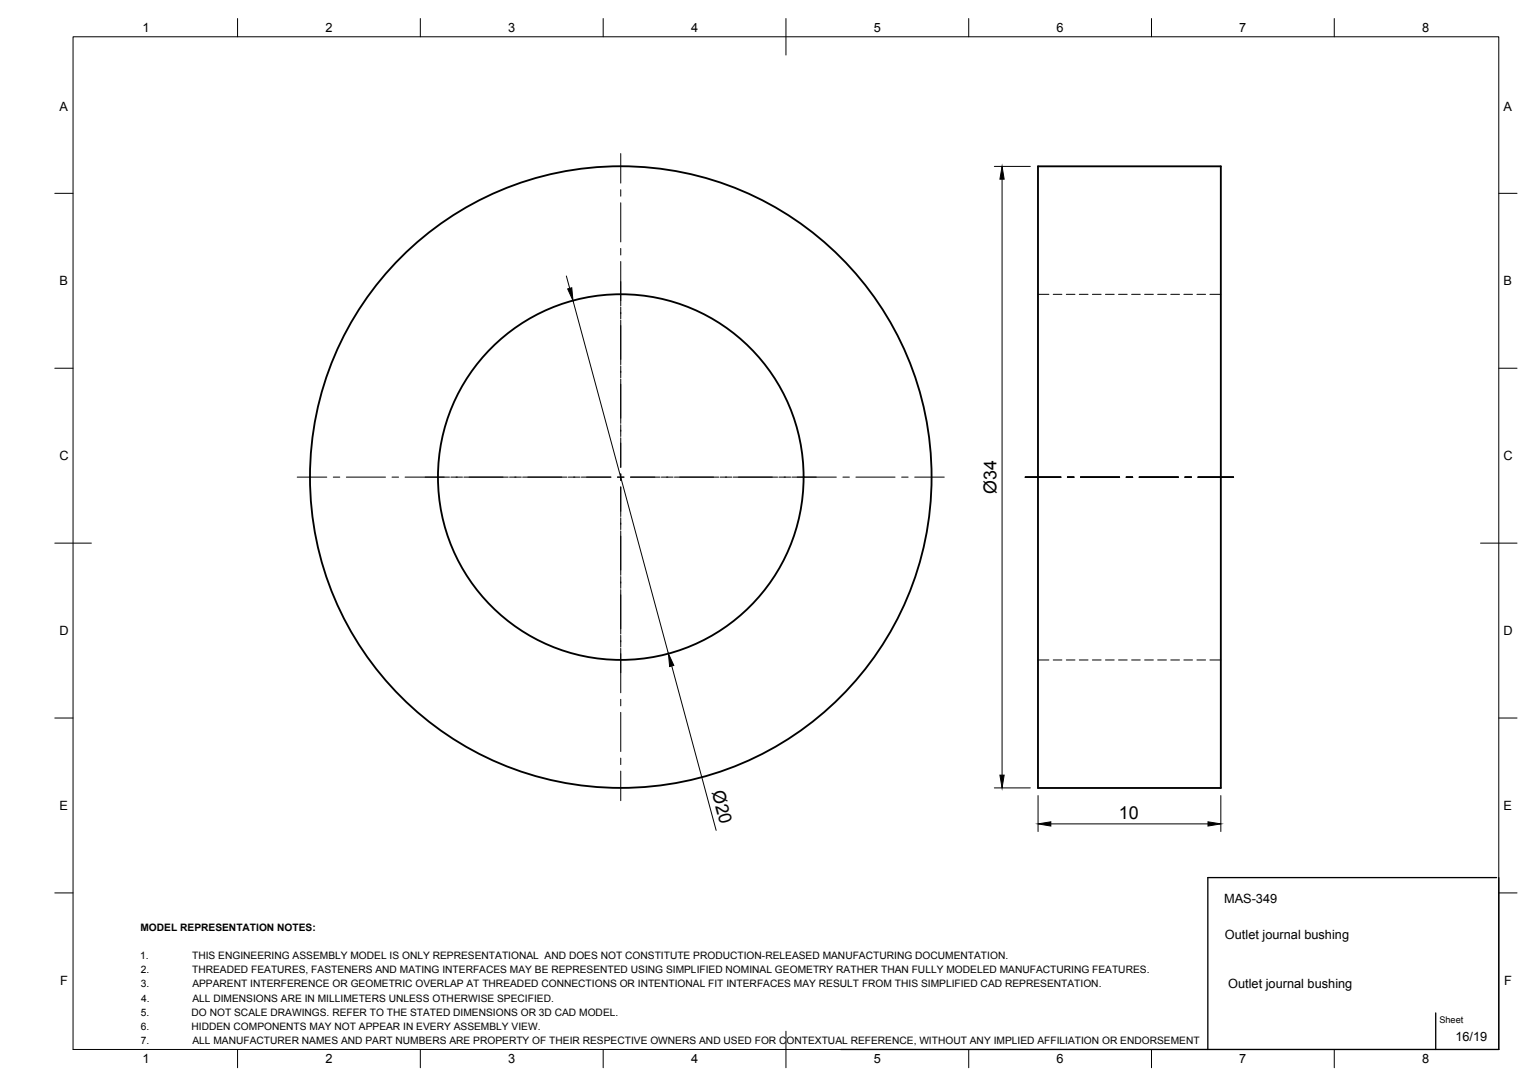
ISO-10303-21;
HEADER;
/* Generated by software containing ST-Developer
 * from STEP Tools, Inc. (www.steptools.com) 
 */

FILE_DESCRIPTION(
/* description */ ('Independent two-stage semi-open centrifugal-pump CAD. Shared impeller
s, open-machinable return casings, removable diaphragms, bronze wear/j
ournal rings, volume-preserving seal instances, retained keyed shaft, 
opposed mechanical face rings and partly threaded tie hardware. Native
 shaft rotation. Geometric topology/clearance only; flow/head/efficien
cy, pressure, cavitation, balance, preload, face loading and secondary
 seal fits/bonds, material/thermal/tolerance selection and life unassi
gned. External drive, coupling, anchors and piping bolts omitted.'),
/* implementation_level */ '2;1');

FILE_NAME(
/* name */ 'Outlet journal bushing.step',
/* time_stamp */ '2026-11-08T18:06:32-08:00',
/* author */ (''),
/* organization */ (''),
/* preprocessor_version */ 'ST-DEVELOPER v20.2',
/* originating_system */ 'Autodesk Translation Framework v15.17.0.0',
/* authorisation */ '');

FILE_SCHEMA (('AUTOMOTIVE_DESIGN { 1 0 10303 214 3 1 1 }'));
ENDSEC;

DATA;
#10=MECHANICAL_DESIGN_GEOMETRIC_PRESENTATION_REPRESENTATION('',(#406),#16687);
#368=SHAPE_REPRESENTATION_RELATIONSHIP('SRR','None',#16777,#387);
#387=ADVANCED_BREP_SHAPE_REPRESENTATION('',(#425),#16681);
#406=STYLED_ITEM('',(#16875),#425);
#425=MANIFOLD_SOLID_BREP('Body1',#6125);
#543=FACE_BOUND('',#1442,.T.);
#544=FACE_BOUND('',#1444,.T.);
#663=PLANE('',#6878);
#664=PLANE('',#6879);
#980=FACE_OUTER_BOUND('',#1439,.T.);
#981=FACE_OUTER_BOUND('',#1440,.T.);
#982=FACE_OUTER_BOUND('',#1441,.T.);
#983=FACE_OUTER_BOUND('',#1443,.T.);
#1439=EDGE_LOOP('',(#5329,#5330,#5331,#5332));
#1440=EDGE_LOOP('',(#5333,#5334,#5335,#5336));
#1441=EDGE_LOOP('',(#5337));
#1442=EDGE_LOOP('',(#5338));
#1443=EDGE_LOOP('',(#5339));
#1444=EDGE_LOOP('',(#5340));
#1820=LINE('',#15192,#2189);
#1821=LINE('',#15198,#2190);
#2189=VECTOR('',#8372,1.);
#2190=VECTOR('',#8379,1.7);
#2470=CIRCLE('',#6873,1.);
#2471=CIRCLE('',#6874,1.);
#2472=CIRCLE('',#6876,1.7);
#2473=CIRCLE('',#6877,1.7);
#2977=VERTEX_POINT('',#15189);
#2978=VERTEX_POINT('',#15191);
#2979=VERTEX_POINT('',#15195);
#2980=VERTEX_POINT('',#15197);
#3774=EDGE_CURVE('',#2977,#2977,#2470,.T.);
#3775=EDGE_CURVE('',#2977,#2978,#1820,.T.);
#3776=EDGE_CURVE('',#2978,#2978,#2471,.T.);
#3777=EDGE_CURVE('',#2979,#2979,#2472,.T.);
#3778=EDGE_CURVE('',#2979,#2980,#1821,.T.);
#3779=EDGE_CURVE('',#2980,#2980,#2473,.T.);
#5329=ORIENTED_EDGE('',*,*,#3774,.F.);
#5330=ORIENTED_EDGE('',*,*,#3775,.T.);
#5331=ORIENTED_EDGE('',*,*,#3776,.T.);
#5332=ORIENTED_EDGE('',*,*,#3775,.F.);
#5333=ORIENTED_EDGE('',*,*,#3777,.F.);
#5334=ORIENTED_EDGE('',*,*,#3778,.T.);
#5335=ORIENTED_EDGE('',*,*,#3779,.T.);
#5336=ORIENTED_EDGE('',*,*,#3778,.F.);
#5337=ORIENTED_EDGE('',*,*,#3777,.T.);
#5338=ORIENTED_EDGE('',*,*,#3774,.T.);
#5339=ORIENTED_EDGE('',*,*,#3779,.F.);
#5340=ORIENTED_EDGE('',*,*,#3776,.F.);
#5738=CYLINDRICAL_SURFACE('',#6872,1.);
#5739=CYLINDRICAL_SURFACE('',#6875,1.7);
#6059=ADVANCED_FACE('',(#980),#5738,.F.);
#6060=ADVANCED_FACE('',(#981),#5739,.T.);
#6061=ADVANCED_FACE('',(#982,#543),#663,.T.);
#6062=ADVANCED_FACE('',(#983,#544),#664,.F.);
#6125=CLOSED_SHELL('',(#6059,#6060,#6061,#6062));
#6871=AXIS2_PLACEMENT_3D('',#15187,#8366,#8367);
#6872=AXIS2_PLACEMENT_3D('',#15188,#8368,#8369);
#6873=AXIS2_PLACEMENT_3D('',#15190,#8370,#8371);
#6874=AXIS2_PLACEMENT_3D('',#15193,#8373,#8374);
#6875=AXIS2_PLACEMENT_3D('',#15194,#8375,#8376);
#6876=AXIS2_PLACEMENT_3D('',#15196,#8377,#8378);
#6877=AXIS2_PLACEMENT_3D('',#15199,#8380,#8381);
#6878=AXIS2_PLACEMENT_3D('',#15200,#8382,#8383);
#6879=AXIS2_PLACEMENT_3D('',#15201,#8384,#8385);
#8366=DIRECTION('axis',(0.,0.,1.));
#8367=DIRECTION('refdir',(1.,0.,0.));
#8368=DIRECTION('center_axis',(0.,0.,1.));
#8369=DIRECTION('ref_axis',(1.,0.,0.));
#8370=DIRECTION('center_axis',(0.,0.,-1.));
#8371=DIRECTION('ref_axis',(1.,0.,0.));
#8372=DIRECTION('',(0.,0.,-1.));
#8373=DIRECTION('center_axis',(0.,0.,-1.));
#8374=DIRECTION('ref_axis',(1.,0.,0.));
#8375=DIRECTION('center_axis',(0.,0.,1.));
#8376=DIRECTION('ref_axis',(1.,0.,0.));
#8377=DIRECTION('center_axis',(0.,0.,1.));
#8378=DIRECTION('ref_axis',(1.,0.,0.));
#8379=DIRECTION('',(0.,0.,-1.));
#8380=DIRECTION('center_axis',(0.,0.,1.));
#8381=DIRECTION('ref_axis',(1.,0.,0.));
#8382=DIRECTION('center_axis',(0.,0.,1.));
#8383=DIRECTION('ref_axis',(1.,0.,0.));
#8384=DIRECTION('center_axis',(0.,0.,1.));
#8385=DIRECTION('ref_axis',(1.,0.,0.));
#15187=CARTESIAN_POINT('',(0.,0.,0.));
#15188=CARTESIAN_POINT('Origin',(0.,0.,0.));
#15189=CARTESIAN_POINT('',(-1.,-1.22464679914735E-16,1.));
#15190=CARTESIAN_POINT('Origin',(0.,0.,1.));
#15191=CARTESIAN_POINT('',(-1.,-1.22464679914735E-16,0.));
#15192=CARTESIAN_POINT('',(-1.,-1.22464679914735E-16,0.));
#15193=CARTESIAN_POINT('Origin',(0.,0.,0.));
#15194=CARTESIAN_POINT('Origin',(0.,0.,0.));
#15195=CARTESIAN_POINT('',(-1.7,-2.0818995585505E-16,1.));
#15196=CARTESIAN_POINT('Origin',(0.,0.,1.));
#15197=CARTESIAN_POINT('',(-1.7,-2.0818995585505E-16,0.));
#15198=CARTESIAN_POINT('',(-1.7,-2.0818995585505E-16,0.));
#15199=CARTESIAN_POINT('Origin',(0.,0.,0.));
#15200=CARTESIAN_POINT('Origin',(0.,0.,1.));
#15201=CARTESIAN_POINT('Origin',(0.,0.,0.));
#16660=UNCERTAINTY_MEASURE_WITH_UNIT(LENGTH_MEASURE(0.001),#16688,
'DISTANCE_ACCURACY_VALUE',
'Maximum model space distance between geometric entities at asserted c
onnectivities');
#16666=UNCERTAINTY_MEASURE_WITH_UNIT(LENGTH_MEASURE(0.001),#16688,
'DISTANCE_ACCURACY_VALUE',
'Maximum model space distance between geometric entities at asserted c
onnectivities');
#16681=(
GEOMETRIC_REPRESENTATION_CONTEXT(3)
GLOBAL_UNCERTAINTY_ASSIGNED_CONTEXT((#16660))
GLOBAL_UNIT_ASSIGNED_CONTEXT((#16688,#16690,#16691))
REPRESENTATION_CONTEXT('','3D')
);
#16687=(
GEOMETRIC_REPRESENTATION_CONTEXT(3)
GLOBAL_UNCERTAINTY_ASSIGNED_CONTEXT((#16666))
GLOBAL_UNIT_ASSIGNED_CONTEXT((#16688,#16690,#16691))
REPRESENTATION_CONTEXT('','3D')
);
#16688=(
LENGTH_UNIT()
NAMED_UNIT(*)
SI_UNIT(.CENTI.,.METRE.)
);
#16690=(
NAMED_UNIT(*)
PLANE_ANGLE_UNIT()
SI_UNIT($,.RADIAN.)
);
#16691=(
NAMED_UNIT(*)
SI_UNIT($,.STERADIAN.)
SOLID_ANGLE_UNIT()
);
#16706=SHAPE_DEFINITION_REPRESENTATION(#16726,#16777);
#16726=PRODUCT_DEFINITION_SHAPE('',$,#16798);
#16777=SHAPE_REPRESENTATION('',(#6871),#16681);
#16783=PRODUCT_DEFINITION_CONTEXT('part definition',#16845,'design');
#16798=PRODUCT_DEFINITION('Outlet journal bushing',
'Outlet journal bushing',#16818,#16783);
#16818=PRODUCT_DEFINITION_FORMATION('',$,#16861);
#16845=APPLICATION_CONTEXT(
'Core Data for Automotive Mechanical Design Process');
#16846=PRODUCT_CONTEXT('part definition',#16845,'mechanical');
#16861=PRODUCT('Outlet journal bushing','Outlet journal bushing',$,(#16846));
#16875=PRESENTATION_STYLE_ASSIGNMENT((#16890));
#16890=SURFACE_STYLE_USAGE(.BOTH.,#16905);
#16905=SURFACE_SIDE_STYLE('',(#16920));
#16920=SURFACE_STYLE_FILL_AREA(#16935);
#16935=FILL_AREA_STYLE('Journal gray',(#16950));
#16950=FILL_AREA_STYLE_COLOUR('Journal gray',#16965);
#16965=COLOUR_RGB('Journal gray',0.725490196078431,0.752941176470588,0.792156862745098);
ENDSEC;
END-ISO-10303-21;
